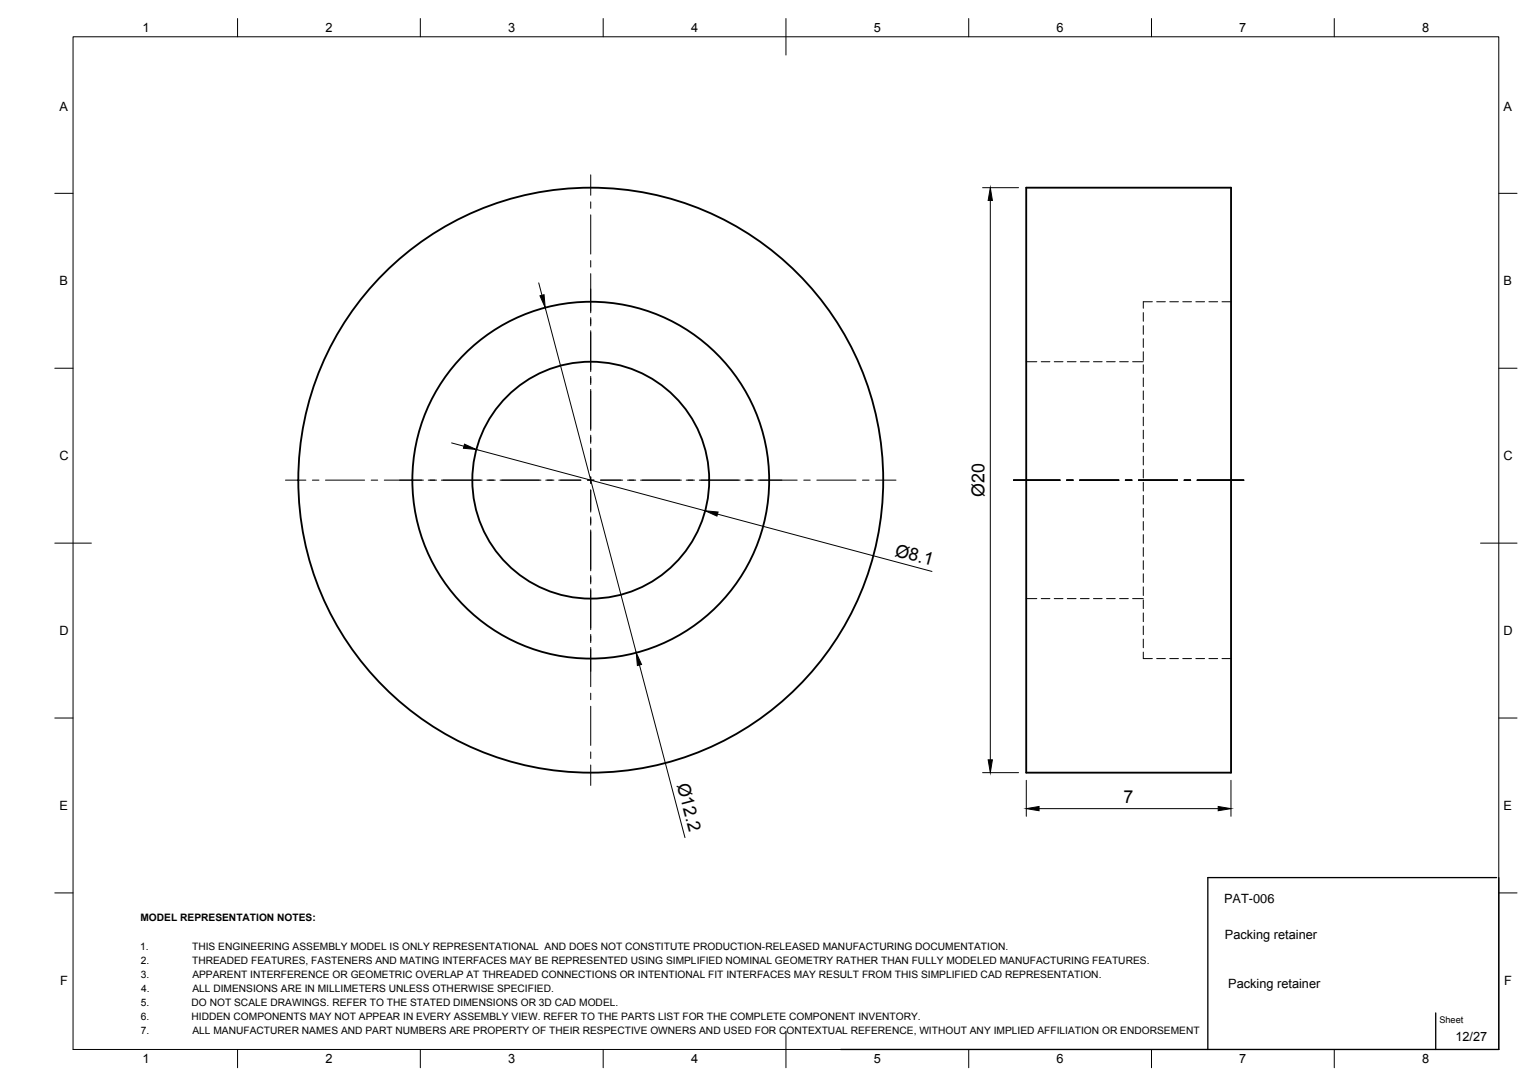
ISO-10303-21;
HEADER;
/* Generated by software containing ST-Developer
 * from STEP Tools, Inc. (www.steptools.com) 
 */

FILE_DESCRIPTION(
/* description */ ('Ball-type isolation valve (generic)'),
/* implementation_level */ '2;1');

FILE_NAME(
/* name */ 'Packing retainer.step',
/* time_stamp */ '2026-10-27T10:53:05-07:00',
/* author */ (''),
/* organization */ (''),
/* preprocessor_version */ 'ST-DEVELOPER v20.2',
/* originating_system */ 'Autodesk Translation Framework v15.17.0.0',
/* authorisation */ '');

FILE_SCHEMA (('AUTOMOTIVE_DESIGN { 1 0 10303 214 3 1 1 }'));
ENDSEC;

DATA;
#10=MECHANICAL_DESIGN_GEOMETRIC_PRESENTATION_REPRESENTATION('',(#284),#7425);
#232=SHAPE_REPRESENTATION_RELATIONSHIP('SRR','None',#7542,#258);
#258=ADVANCED_BREP_SHAPE_REPRESENTATION('',(#310),#7405);
#284=STYLED_ITEM('',(#7730),#310);
#310=MANIFOLD_SOLID_BREP('Body1',#4089);
#376=FACE_BOUND('',#950,.T.);
#377=FACE_BOUND('',#954,.T.);
#378=FACE_BOUND('',#956,.T.);
#459=PLANE('',#4556);
#460=PLANE('',#4563);
#461=PLANE('',#4564);
#654=FACE_OUTER_BOUND('',#948,.T.);
#655=FACE_OUTER_BOUND('',#949,.T.);
#656=FACE_OUTER_BOUND('',#951,.T.);
#657=FACE_OUTER_BOUND('',#952,.T.);
#658=FACE_OUTER_BOUND('',#953,.T.);
#659=FACE_OUTER_BOUND('',#955,.T.);
#948=EDGE_LOOP('',(#3093,#3094,#3095,#3096));
#949=EDGE_LOOP('',(#3097));
#950=EDGE_LOOP('',(#3098));
#951=EDGE_LOOP('',(#3099,#3100,#3101,#3102));
#952=EDGE_LOOP('',(#3103,#3104,#3105,#3106));
#953=EDGE_LOOP('',(#3107));
#954=EDGE_LOOP('',(#3108));
#955=EDGE_LOOP('',(#3109));
#956=EDGE_LOOP('',(#3110));
#1254=LINE('',#6555,#1562);
#1255=LINE('',#6563,#1563);
#1256=LINE('',#6568,#1564);
#1562=VECTOR('',#5299,0.61);
#1563=VECTOR('',#5310,0.405);
#1564=VECTOR('',#5315,1.);
#1851=CIRCLE('',#4554,0.61);
#1852=CIRCLE('',#4555,0.61);
#1853=CIRCLE('',#4557,0.405);
#1854=CIRCLE('',#4559,0.405);
#1855=CIRCLE('',#4561,1.);
#1856=CIRCLE('',#4562,1.);
#2063=VERTEX_POINT('',#6552);
#2064=VERTEX_POINT('',#6554);
#2065=VERTEX_POINT('',#6558);
#2066=VERTEX_POINT('',#6561);
#2067=VERTEX_POINT('',#6565);
#2068=VERTEX_POINT('',#6567);
#2439=EDGE_CURVE('',#2063,#2063,#1851,.T.);
#2440=EDGE_CURVE('',#2063,#2064,#1254,.T.);
#2441=EDGE_CURVE('',#2064,#2064,#1852,.T.);
#2442=EDGE_CURVE('',#2065,#2065,#1853,.T.);
#2443=EDGE_CURVE('',#2066,#2066,#1854,.T.);
#2444=EDGE_CURVE('',#2066,#2065,#1255,.T.);
#2445=EDGE_CURVE('',#2067,#2067,#1855,.T.);
#2446=EDGE_CURVE('',#2067,#2068,#1256,.T.);
#2447=EDGE_CURVE('',#2068,#2068,#1856,.T.);
#3093=ORIENTED_EDGE('',*,*,#2439,.F.);
#3094=ORIENTED_EDGE('',*,*,#2440,.T.);
#3095=ORIENTED_EDGE('',*,*,#2441,.T.);
#3096=ORIENTED_EDGE('',*,*,#2440,.F.);
#3097=ORIENTED_EDGE('',*,*,#2441,.F.);
#3098=ORIENTED_EDGE('',*,*,#2442,.F.);
#3099=ORIENTED_EDGE('',*,*,#2443,.F.);
#3100=ORIENTED_EDGE('',*,*,#2444,.T.);
#3101=ORIENTED_EDGE('',*,*,#2442,.T.);
#3102=ORIENTED_EDGE('',*,*,#2444,.F.);
#3103=ORIENTED_EDGE('',*,*,#2445,.F.);
#3104=ORIENTED_EDGE('',*,*,#2446,.T.);
#3105=ORIENTED_EDGE('',*,*,#2447,.T.);
#3106=ORIENTED_EDGE('',*,*,#2446,.F.);
#3107=ORIENTED_EDGE('',*,*,#2445,.T.);
#3108=ORIENTED_EDGE('',*,*,#2443,.T.);
#3109=ORIENTED_EDGE('',*,*,#2447,.F.);
#3110=ORIENTED_EDGE('',*,*,#2439,.T.);
#3795=CYLINDRICAL_SURFACE('',#4553,0.61);
#3796=CYLINDRICAL_SURFACE('',#4558,0.405);
#3797=CYLINDRICAL_SURFACE('',#4560,1.);
#3908=ADVANCED_FACE('',(#654),#3795,.F.);
#3909=ADVANCED_FACE('',(#655,#376),#459,.F.);
#3910=ADVANCED_FACE('',(#656),#3796,.F.);
#3911=ADVANCED_FACE('',(#657),#3797,.T.);
#3912=ADVANCED_FACE('',(#658,#377),#460,.T.);
#3913=ADVANCED_FACE('',(#659,#378),#461,.F.);
#4089=CLOSED_SHELL('',(#3908,#3909,#3910,#3911,#3912,#3913));
#4552=AXIS2_PLACEMENT_3D('',#6550,#5293,#5294);
#4553=AXIS2_PLACEMENT_3D('',#6551,#5295,#5296);
#4554=AXIS2_PLACEMENT_3D('',#6553,#5297,#5298);
#4555=AXIS2_PLACEMENT_3D('',#6556,#5300,#5301);
#4556=AXIS2_PLACEMENT_3D('',#6557,#5302,#5303);
#4557=AXIS2_PLACEMENT_3D('',#6559,#5304,#5305);
#4558=AXIS2_PLACEMENT_3D('',#6560,#5306,#5307);
#4559=AXIS2_PLACEMENT_3D('',#6562,#5308,#5309);
#4560=AXIS2_PLACEMENT_3D('',#6564,#5311,#5312);
#4561=AXIS2_PLACEMENT_3D('',#6566,#5313,#5314);
#4562=AXIS2_PLACEMENT_3D('',#6569,#5316,#5317);
#4563=AXIS2_PLACEMENT_3D('',#6570,#5318,#5319);
#4564=AXIS2_PLACEMENT_3D('',#6571,#5320,#5321);
#5293=DIRECTION('axis',(0.,0.,1.));
#5294=DIRECTION('refdir',(1.,0.,0.));
#5295=DIRECTION('center_axis',(0.,0.,1.));
#5296=DIRECTION('ref_axis',(1.,0.,0.));
#5297=DIRECTION('center_axis',(0.,0.,1.));
#5298=DIRECTION('ref_axis',(1.,0.,0.));
#5299=DIRECTION('',(0.,0.,1.));
#5300=DIRECTION('center_axis',(0.,0.,1.));
#5301=DIRECTION('ref_axis',(1.,0.,0.));
#5302=DIRECTION('center_axis',(0.,0.,1.));
#5303=DIRECTION('ref_axis',(1.,0.,0.));
#5304=DIRECTION('center_axis',(0.,0.,-1.));
#5305=DIRECTION('ref_axis',(1.,0.,0.));
#5306=DIRECTION('center_axis',(0.,0.,1.));
#5307=DIRECTION('ref_axis',(1.,0.,0.));
#5308=DIRECTION('center_axis',(0.,0.,-1.));
#5309=DIRECTION('ref_axis',(1.,0.,0.));
#5310=DIRECTION('',(0.,0.,-1.));
#5311=DIRECTION('center_axis',(0.,0.,1.));
#5312=DIRECTION('ref_axis',(1.,0.,0.));
#5313=DIRECTION('center_axis',(0.,0.,1.));
#5314=DIRECTION('ref_axis',(1.,0.,0.));
#5315=DIRECTION('',(0.,0.,-1.));
#5316=DIRECTION('center_axis',(0.,0.,1.));
#5317=DIRECTION('ref_axis',(1.,0.,0.));
#5318=DIRECTION('center_axis',(0.,0.,1.));
#5319=DIRECTION('ref_axis',(1.,0.,0.));
#5320=DIRECTION('center_axis',(0.,0.,1.));
#5321=DIRECTION('ref_axis',(1.,0.,0.));
#6550=CARTESIAN_POINT('',(0.,0.,0.));
#6551=CARTESIAN_POINT('Origin',(0.,0.,7.9));
#6552=CARTESIAN_POINT('',(-0.61,-7.47034547479885E-17,8.));
#6553=CARTESIAN_POINT('Origin',(0.,0.,8.));
#6554=CARTESIAN_POINT('',(-0.61,-7.47034547479885E-17,8.3));
#6555=CARTESIAN_POINT('',(-0.61,-7.47034547479885E-17,7.9));
#6556=CARTESIAN_POINT('Origin',(0.,0.,8.3));
#6557=CARTESIAN_POINT('Origin',(0.,0.,8.3));
#6558=CARTESIAN_POINT('',(-0.405,4.95981953654678E-17,8.3));
#6559=CARTESIAN_POINT('Origin',(0.,0.,8.3));
#6560=CARTESIAN_POINT('Origin',(0.,0.,8.));
#6561=CARTESIAN_POINT('',(-0.405,-4.95981953654678E-17,8.7));
#6562=CARTESIAN_POINT('Origin',(0.,0.,8.7));
#6563=CARTESIAN_POINT('',(-0.405,-4.95981953654678E-17,8.));
#6564=CARTESIAN_POINT('Origin',(0.,0.,8.));
#6565=CARTESIAN_POINT('',(-1.,-1.22464679914735E-16,8.7));
#6566=CARTESIAN_POINT('Origin',(0.,0.,8.7));
#6567=CARTESIAN_POINT('',(-1.,-1.22464679914735E-16,8.));
#6568=CARTESIAN_POINT('',(-1.,-1.22464679914735E-16,8.));
#6569=CARTESIAN_POINT('Origin',(0.,0.,8.));
#6570=CARTESIAN_POINT('Origin',(0.,0.,8.7));
#6571=CARTESIAN_POINT('Origin',(0.,0.,8.));
#7375=UNCERTAINTY_MEASURE_WITH_UNIT(LENGTH_MEASURE(0.001),#7426,
'DISTANCE_ACCURACY_VALUE',
'Maximum model space distance between geometric entities at asserted c
onnectivities');
#7395=UNCERTAINTY_MEASURE_WITH_UNIT(LENGTH_MEASURE(0.001),#7426,
'DISTANCE_ACCURACY_VALUE',
'Maximum model space distance between geometric entities at asserted c
onnectivities');
#7405=(
GEOMETRIC_REPRESENTATION_CONTEXT(3)
GLOBAL_UNCERTAINTY_ASSIGNED_CONTEXT((#7375))
GLOBAL_UNIT_ASSIGNED_CONTEXT((#7426,#7428,#7429))
REPRESENTATION_CONTEXT('','3D')
);
#7425=(
GEOMETRIC_REPRESENTATION_CONTEXT(3)
GLOBAL_UNCERTAINTY_ASSIGNED_CONTEXT((#7395))
GLOBAL_UNIT_ASSIGNED_CONTEXT((#7426,#7428,#7429))
REPRESENTATION_CONTEXT('','3D')
);
#7426=(
LENGTH_UNIT()
NAMED_UNIT(*)
SI_UNIT(.CENTI.,.METRE.)
);
#7428=(
NAMED_UNIT(*)
PLANE_ANGLE_UNIT()
SI_UNIT($,.RADIAN.)
);
#7429=(
NAMED_UNIT(*)
SI_UNIT($,.STERADIAN.)
SOLID_ANGLE_UNIT()
);
#7439=SHAPE_DEFINITION_REPRESENTATION(#7468,#7542);
#7468=PRODUCT_DEFINITION_SHAPE('',$,#7572);
#7542=SHAPE_REPRESENTATION('',(#4552),#7405);
#7562=PRODUCT_DEFINITION_CONTEXT('part definition',#7651,'design');
#7572=PRODUCT_DEFINITION('Packing retainer','Packing retainer',#7601,#7562);
#7601=PRODUCT_DEFINITION_FORMATION('',$,#7662);
#7651=APPLICATION_CONTEXT(
'Core Data for Automotive Mechanical Design Process');
#7652=PRODUCT_CONTEXT('part definition',#7651,'mechanical');
#7662=PRODUCT('Packing retainer','Packing retainer','Packing retainer',
(#7652));
#7724=COLOUR_RGB('Light Blue',0.38,0.62,0.78);
#7725=FILL_AREA_STYLE_COLOUR('',#7724);
#7726=FILL_AREA_STYLE('',(#7725));
#7727=SURFACE_STYLE_FILL_AREA(#7726);
#7728=SURFACE_SIDE_STYLE('',(#7727));
#7729=SURFACE_STYLE_USAGE(.BOTH.,#7728);
#7730=PRESENTATION_STYLE_ASSIGNMENT((#7729));
ENDSEC;
END-ISO-10303-21;
